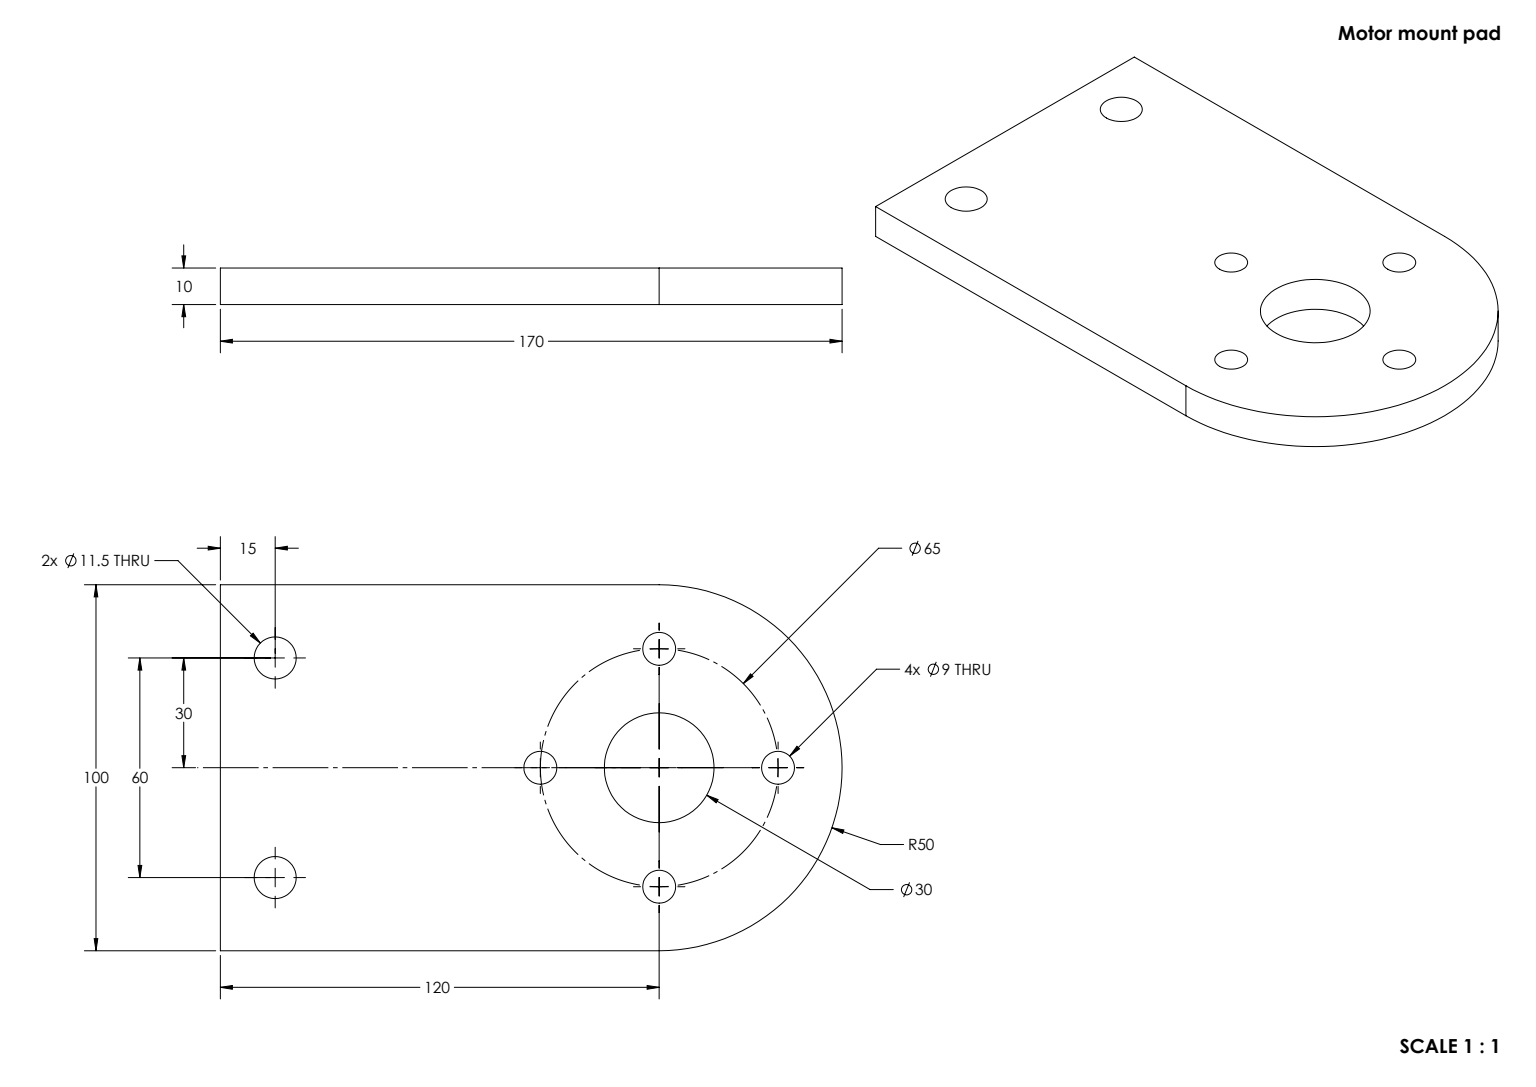
ISO-10303-21;
HEADER;
FILE_DESCRIPTION (('STEP AP214'),
    '1' );
FILE_NAME ('Motor mount pad.step',
    '2026-10-24T15:53:57',
    ( '' ),
    ( '' ),
    'SwSTEP 2.0',
    'SolidWorks 2025',
    '' );
FILE_SCHEMA (( 'AUTOMOTIVE_DESIGN' ));
ENDSEC;

DATA;
#1=CARTESIAN_POINT ( 'NONE',  ( -86.99999999999945999, 120.0000000000003126, 10.00000000000000888 ) ) ;
#4=FACE_BOUND ( 'NONE', #3829, .T. ) ;
#59=DIRECTION ( 'NONE',  ( 3.919652622816902408E-30, 3.944304526105059027E-30, -1.000000000000000000 ) ) ;
#65=LINE ( 'NONE', #1952, #3706 ) ;
#75=DIRECTION ( 'NONE',  ( -3.919652622816902408E-30, -3.944304526105059027E-30, 1.000000000000000000 ) ) ;
#91=DIRECTION ( 'NONE',  ( -3.919652622816902408E-30, -3.944304526105059027E-30, 1.000000000000000000 ) ) ;
#98=EDGE_CURVE ( 'NONE', #113, #2214, #3687, .T. ) ;
#105=UNCERTAINTY_MEASURE_WITH_UNIT (LENGTH_MEASURE( 1.000000000000000082E-05 ), #1753, 'distance_accuracy_value', 'NONE');
#109=DIRECTION ( 'NONE',  ( 3.919652622816902408E-30, 3.944304526105059027E-30, -1.000000000000000000 ) ) ;
#113=VERTEX_POINT ( 'NONE', #6673 ) ;
#117=ORIENTED_EDGE ( 'NONE', *, *, #6294, .F. ) ;
#136=DIRECTION ( 'NONE',  ( -3.919652622816902408E-30, -3.944304526105059027E-30, 1.000000000000000000 ) ) ;
#142=ORIENTED_EDGE ( 'NONE', *, *, #672, .F. ) ;
#165=EDGE_CURVE ( 'NONE', #2264, #3370, #4990, .T. ) ;
#167=CARTESIAN_POINT ( 'NONE',  ( -99.99999999999961631, 120.0000000000001137, 10.00000000000000888 ) ) ;
#175=ORIENTED_EDGE ( 'NONE', *, *, #1489, .T. ) ;
#178=VECTOR ( 'NONE', #4210, 1000.000000000000000 ) ;
#217=VECTOR ( 'NONE', #7393, 1000.000000000000000 ) ;
#237=DIRECTION ( 'NONE',  ( -3.919652622816902408E-30, -3.944304526105059027E-30, 1.000000000000000000 ) ) ;
#246=CARTESIAN_POINT ( 'NONE',  ( -86.99999999999944578, 120.0000000000003126, 10.00000000000000888 ) ) ;
#265=AXIS2_PLACEMENT_3D ( 'NONE', #591, #6694, #3898 ) ;
#270=EDGE_LOOP ( 'NONE', ( #1206, #6558, #6515, #500 ) ) ;
#292=DIRECTION ( 'NONE',  ( 1.000000000000000000, 2.715219353702832714E-15, 0.000000000000000000 ) ) ;
#305=VECTOR ( 'NONE', #380, 1000.000000000000000 ) ;
#306=EDGE_CURVE ( 'NONE', #6636, #757, #6561, .T. ) ;
#320=AXIS2_PLACEMENT_3D ( 'NONE', #2121, #5234, #1317 ) ;
#328=DIRECTION ( 'NONE',  ( 3.919652622816902408E-30, 3.944304526105059027E-30, -1.000000000000000000 ) ) ;
#336=AXIS2_PLACEMENT_3D ( 'NONE', #6289, #351, #5640 ) ;
#337=CARTESIAN_POINT ( 'NONE',  ( 0.000000000000000000, 0.000000000000000000, 10.00000000000000888 ) ) ;
#351=DIRECTION ( 'NONE',  ( -3.919652622816902408E-30, -3.944304526105059027E-30, 1.000000000000000000 ) ) ;
#357=UNCERTAINTY_MEASURE_WITH_UNIT (LENGTH_MEASURE( 1.000000000000000082E-05 ), #6514, 'distance_accuracy_value', 'NONE');
#365=CARTESIAN_POINT ( 'NONE',  ( -99.99999999999972999, 0.000000000000000000, 9.999999999999980460 ) ) ;
#377=ORIENTED_EDGE ( 'NONE', *, *, #1254, .F. ) ;
#380=DIRECTION ( 'NONE',  ( -1.619075244245011540E-15, -1.000000000000000000, 3.747089299799789961E-30 ) ) ;
#381=ORIENTED_EDGE ( 'NONE', *, *, #1415, .T. ) ;
#407=AXIS2_PLACEMENT_3D ( 'NONE', #5310, #7916, #3997 ) ;
#419=EDGE_LOOP ( 'NONE', ( #3396, #2400 ) ) ;
#427=VECTOR ( 'NONE', #3150, 1000.000000000000000 ) ;
#437=DIRECTION ( 'NONE',  ( -1.000000000000000000, -2.775557561562916200E-15, 0.000000000000000000 ) ) ;
#439=ADVANCED_FACE ( 'NONE', ( #590 ), #6765, .F. ) ;
#461=CIRCLE ( 'NONE', #2535, 4.499999999999993783 ) ;
#472=FACE_OUTER_BOUND ( 'NONE', #4653, .T. ) ;
#484=VERTEX_POINT ( 'NONE', #6614 ) ;
#486=ORIENTED_EDGE ( 'NONE', *, *, #7335, .T. ) ;
#492=CARTESIAN_POINT ( 'NONE',  ( -14.24999999999983125, 15.00000000000014211, 10.00000000000000888 ) ) ;
#500=ORIENTED_EDGE ( 'NONE', *, *, #647, .F. ) ;
#506=LINE ( 'NONE', #337, #7415 ) ;
#522=ADVANCED_FACE ( 'NONE', ( #8225 ), #7611, .F. ) ;
#548=CIRCLE ( 'NONE', #5427, 4.499999999999983125 ) ;
#573=DIRECTION ( 'NONE',  ( 3.919652622816902408E-30, 3.944304526105059027E-30, -1.000000000000000000 ) ) ;
#575=CARTESIAN_POINT ( 'NONE',  ( -45.49999999999968026, 87.50000000000036948, -1.942890293094023693E-13 ) ) ;
#590=FACE_OUTER_BOUND ( 'NONE', #2757, .T. ) ;
#591=CARTESIAN_POINT ( 'NONE',  ( -82.49999999999945999, 120.0000000000003268, 10.00000000000000888 ) ) ;
#605=VERTEX_POINT ( 'NONE', #5445 ) ;
#639=PLANE ( 'NONE',  #6979 ) ;
#642=AXIS2_PLACEMENT_3D ( 'NONE', #2902, #2253, #6469 ) ;
#647=EDGE_CURVE ( 'NONE', #2499, #2290, #7527, .T. ) ;
#657=DIRECTION ( 'NONE',  ( 3.919652622816902408E-30, 3.944304526105059027E-30, -1.000000000000000000 ) ) ;
#658=CARTESIAN_POINT ( 'NONE',  ( -82.49999999999945999, 120.0000000000003268, 10.00000000000000888 ) ) ;
#659=AXIS2_PLACEMENT_3D ( 'NONE', #2516, #3903, #4518 ) ;
#672=EDGE_CURVE ( 'NONE', #704, #605, #506, .T. ) ;
#683=VERTEX_POINT ( 'NONE', #6965 ) ;
#694=DIRECTION ( 'NONE',  ( -3.919652622816902408E-30, -3.944304526105059027E-30, 1.000000000000000000 ) ) ;
#704=VERTEX_POINT ( 'NONE', #8349 ) ;
#709=SHAPE_DEFINITION_REPRESENTATION ( #3889, #7270 ) ;
#717=DIRECTION ( 'NONE',  ( 2.775557561562879124E-15, 1.000000000000000000, 3.944304526105070237E-30 ) ) ;
#727=FACE_BOUND ( 'NONE', #4525, .T. ) ;
#739=AXIS2_PLACEMENT_3D ( 'NONE', #6687, #717, #91 ) ;
#751=DIRECTION ( 'NONE',  ( 3.919652622816902408E-30, 3.944304526105059027E-30, -1.000000000000000000 ) ) ;
#757=VERTEX_POINT ( 'NONE', #938 ) ;
#776=DIRECTION ( 'NONE',  ( -3.919652622816902408E-30, -3.944304526105059027E-30, 1.000000000000000000 ) ) ;
#777=DIRECTION ( 'NONE',  ( -1.000000000000000000, 3.498359009886547695E-15, 3.722437396511637546E-30 ) ) ;
#795=EDGE_CURVE ( 'NONE', #2499, #6000, #4916, .T. ) ;
#807=ORIENTED_EDGE ( 'NONE', *, *, #3230, .F. ) ;
#827=CARTESIAN_POINT ( 'NONE',  ( -19.99999999999982947, 15.00000000000012434, 10.00000000000000888 ) ) ;
#886=DIRECTION ( 'NONE',  ( 3.919652622816902408E-30, 3.944304526105059027E-30, -1.000000000000000000 ) ) ;
#910=LINE ( 'NONE', #246, #1515 ) ;
#911=AXIS2_PLACEMENT_3D ( 'NONE', #3791, #7747, #7669 ) ;
#938=CARTESIAN_POINT ( 'NONE',  ( -45.49999999999950262, 152.5000000000003126, -1.942890293094023693E-13 ) ) ;
#952=EDGE_CURVE ( 'NONE', #2264, #484, #8525, .T. ) ;
#989=VECTOR ( 'NONE', #3365, 1000.000000000000000 ) ;
#1000=DIRECTION ( 'NONE',  ( -3.919652622816902408E-30, -3.944304526105059027E-30, 1.000000000000000000 ) ) ;
#1026=AXIS2_PLACEMENT_3D ( 'NONE', #1779, #2283, #6452 ) ;
#1032=EDGE_LOOP ( 'NONE', ( #1487, #8169 ) ) ;
#1104=CARTESIAN_POINT ( 'NONE',  ( -49.99999999999963762, 87.50000000000035527, 9.999999999999786837 ) ) ;
#1107=CARTESIAN_POINT ( 'NONE',  ( -25.74999999999981526, 15.00000000000010836, 10.00000000000000888 ) ) ;
#1119=DIRECTION ( 'NONE',  ( 3.919652622816902408E-30, 3.944304526105059027E-30, -1.000000000000000000 ) ) ;
#1130=CARTESIAN_POINT ( 'NONE',  ( -86.99999999999943157, 120.0000000000003126, -2.775557561562893244E-14 ) ) ;
#1157=CARTESIAN_POINT ( 'NONE',  ( -45.49999999999963052, 87.50000000000036948, 9.999999999999786837 ) ) ;
#1186=ORIENTED_EDGE ( 'NONE', *, *, #2194, .F. ) ;
#1194=CARTESIAN_POINT ( 'NONE',  ( -49.99999999999949551, 152.5000000000003126, -1.942890293094023946E-13 ) ) ;
#1197=DIRECTION ( 'NONE',  ( 1.619075244245011343E-15, 1.000000000000000000, -3.845696912952415736E-30 ) ) ;
#1206=ORIENTED_EDGE ( 'NONE', *, *, #795, .T. ) ;
#1227=EDGE_CURVE ( 'NONE', #4883, #4829, #1432, .T. ) ;
#1254=EDGE_CURVE ( 'NONE', #1438, #6198, #65, .T. ) ;
#1263=ORIENTED_EDGE ( 'NONE', *, *, #2548, .T. ) ;
#1271=ORIENTED_EDGE ( 'NONE', *, *, #7626, .T. ) ;
#1290=FACE_BOUND ( 'NONE', #1032, .T. ) ;
#1299=VECTOR ( 'NONE', #5348, 1000.000000000000000 ) ;
#1302=EDGE_CURVE ( 'NONE', #7833, #7189, #3565, .T. ) ;
#1317=DIRECTION ( 'NONE',  ( 1.000000000000000000, 3.083952846180992055E-15, 0.000000000000000000 ) ) ;
#1323=CYLINDRICAL_SURFACE ( 'NONE', #4448, 4.499999999999990230 ) ;
#1336=FACE_BOUND ( 'NONE', #5358, .T. ) ;
#1346=FACE_OUTER_BOUND ( 'NONE', #4606, .T. ) ;
#1347=ORIENTED_EDGE ( 'NONE', *, *, #4480, .F. ) ;
#1354=CARTESIAN_POINT ( 'NONE',  ( -54.49999999999943867, 152.5000000000003126, 9.999999999999786837 ) ) ;
#1365=ORIENTED_EDGE ( 'NONE', *, *, #7801, .T. ) ;
#1370=CARTESIAN_POINT ( 'NONE',  ( -49.99999999999968026, 87.50000000000035527, -1.942890293094023946E-13 ) ) ;
#1400=AXIS2_PLACEMENT_3D ( 'NONE', #2758, #136, #2163 ) ;
#1404=VECTOR ( 'NONE', #4018, 1000.000000000000000 ) ;
#1415=EDGE_CURVE ( 'NONE', #113, #6113, #8014, .T. ) ;
#1432=LINE ( 'NONE', #6755, #217 ) ;
#1435=CARTESIAN_POINT ( 'NONE',  ( -49.99999999999963762, 87.50000000000035527, 9.999999999999786837 ) ) ;
#1438=VERTEX_POINT ( 'NONE', #6151 ) ;
#1447=ORIENTED_EDGE ( 'NONE', *, *, #7891, .T. ) ;
#1456=DIRECTION ( 'NONE',  ( -1.000000000000000000, -3.083952846180997183E-15, 0.000000000000000000 ) ) ;
#1475=CYLINDRICAL_SURFACE ( 'NONE', #3816, 5.749999999999984013 ) ;
#1484=CARTESIAN_POINT ( 'NONE',  ( -49.99999999999944578, 152.5000000000003126, 9.999999999999786837 ) ) ;
#1487=ORIENTED_EDGE ( 'NONE', *, *, #1489, .F. ) ;
#1489=EDGE_CURVE ( 'NONE', #1438, #4229, #7320, .T. ) ;
#1515=VECTOR ( 'NONE', #2255, 1000.000000000000000 ) ;
#1517=ORIENTED_EDGE ( 'NONE', *, *, #7484, .T. ) ;
#1527=AXIS2_PLACEMENT_3D ( 'NONE', #8120, #6818, #2275 ) ;
#1535=ORIENTED_EDGE ( 'NONE', *, *, #306, .T. ) ;
#1550=CARTESIAN_POINT ( 'NONE',  ( -85.74999999999980105, 15.00000000000010836, 10.00000000000017586 ) ) ;
#1564=ORIENTED_EDGE ( 'NONE', *, *, #8209, .T. ) ;
#1569=LINE ( 'NONE', #2114, #8262 ) ;
#1607=EDGE_LOOP ( 'NONE', ( #1271, #142, #5458, #2317 ) ) ;
#1626=EDGE_CURVE ( 'NONE', #5659, #5363, #2315, .T. ) ;
#1629=CARTESIAN_POINT ( 'NONE',  ( -19.99999999999986855, 15.00000000000012434, 0.000000000000000000 ) ) ;
#1633=DIRECTION ( 'NONE',  ( 3.919652622816902408E-30, 3.944304526105059027E-30, -1.000000000000000000 ) ) ;
#1641=CARTESIAN_POINT ( 'NONE',  ( -54.49999999999948841, 152.5000000000003126, -1.942890293094024198E-13 ) ) ;
#1650=VERTEX_POINT ( 'NONE', #1 ) ;
#1686=VECTOR ( 'NONE', #7251, 1000.000000000000000 ) ;
#1700=CIRCLE ( 'NONE', #5625, 4.499999999999983125 ) ;
#1706=EDGE_LOOP ( 'NONE', ( #2673, #1263, #5085, #5047 ) ) ;
#1711=AXIS2_PLACEMENT_3D ( 'NONE', #8438, #7050, #1197 ) ;
#1732=ORIENTED_EDGE ( 'NONE', *, *, #3516, .T. ) ;
#1752=DIRECTION ( 'NONE',  ( 3.919652622816902408E-30, 3.944304526105059027E-30, -1.000000000000000000 ) ) ;
#1753=( LENGTH_UNIT ( ) NAMED_UNIT ( * ) SI_UNIT ( .MILLI., .METRE. ) );
#1779=CARTESIAN_POINT ( 'NONE',  ( -79.99999999999980105, 15.00000000000012434, 10.00000000000017586 ) ) ;
#1788=CARTESIAN_POINT ( 'NONE',  ( -49.99999999999953815, 120.0000000000003268, 9.999999999999980460 ) ) ;
#1803=DIRECTION ( 'NONE',  ( 3.919652622816902408E-30, 3.944304526105059027E-30, -1.000000000000000000 ) ) ;
#1867=DIRECTION ( 'NONE',  ( -3.919652622816902408E-30, -3.944304526105059027E-30, 1.000000000000000000 ) ) ;
#1881=AXIS2_PLACEMENT_3D ( 'NONE', #2639, #4555, #7817 ) ;
#1883=DIRECTION ( 'NONE',  ( 3.919652622816902408E-30, 3.944304526105059027E-30, -1.000000000000000000 ) ) ;
#1892=AXIS2_PLACEMENT_3D ( 'NONE', #6921, #776, #2136 ) ;
#1903=CIRCLE ( 'NONE', #3449, 5.749999999999985789 ) ;
#1920=DIRECTION ( 'NONE',  ( 3.919652622816902408E-30, 3.944304526105059027E-30, -1.000000000000000000 ) ) ;
#1952=CARTESIAN_POINT ( 'NONE',  ( -21.99999999999954881, 120.0000000000003126, 9.999999999999980460 ) ) ;
#1995=CARTESIAN_POINT ( 'NONE',  ( -49.99999999999968026, 87.50000000000035527, -1.942890293094023946E-13 ) ) ;
#2017=ADVANCED_FACE ( 'NONE', ( #5749 ), #3645, .F. ) ;
#2089=CIRCLE ( 'NONE', #8200, 14.99999999999987388 ) ;
#2102=CARTESIAN_POINT ( 'NONE',  ( -17.49999999999955236, 120.0000000000003268, 9.999999999999980460 ) ) ;
#2110=AXIS2_PLACEMENT_3D ( 'NONE', #3460, #2803, #2846 ) ;
#2114=CARTESIAN_POINT ( 'NONE',  ( -99.99999999999961631, 120.0000000000001137, 10.00000000000000888 ) ) ;
#2116=ORIENTED_EDGE ( 'NONE', *, *, #7710, .F. ) ;
#2121=CARTESIAN_POINT ( 'NONE',  ( -49.99999999999963762, 87.50000000000035527, 9.999999999999786837 ) ) ;
#2136=DIRECTION ( 'NONE',  ( 1.000000000000000000, 3.083952846180994816E-15, -3.821045009664285742E-30 ) ) ;
#2152=ORIENTED_EDGE ( 'NONE', *, *, #7413, .T. ) ;
#2163=DIRECTION ( 'NONE',  ( 1.000000000000000000, 2.715219353702835081E-15, -3.821045009664285041E-30 ) ) ;
#2166=ADVANCED_FACE ( 'NONE', ( #4634 ), #7846, .F. ) ;
#2168=DIRECTION ( 'NONE',  ( 3.919652622816902408E-30, 3.944304526105059027E-30, -1.000000000000000000 ) ) ;
#2169=CIRCLE ( 'NONE', #911, 49.99999999999998579 ) ;
#2173=CARTESIAN_POINT ( 'NONE',  ( -49.99999999999953815, 120.0000000000003268, 9.999999999999980460 ) ) ;
#2175=FACE_OUTER_BOUND ( 'NONE', #5707, .T. ) ;
#2183=LINE ( 'NONE', #4137, #305 ) ;
#2194=EDGE_CURVE ( 'NONE', #6000, #3126, #6856, .T. ) ;
#2214=VERTEX_POINT ( 'NONE', #6727 ) ;
#2216=VERTEX_POINT ( 'NONE', #3412 ) ;
#2244=DIRECTION ( 'NONE',  ( -3.919652622816902408E-30, -3.944304526105059027E-30, 1.000000000000000000 ) ) ;
#2253=DIRECTION ( 'NONE',  ( -3.919652622816902408E-30, -3.944304526105059027E-30, 1.000000000000000000 ) ) ;
#2255=DIRECTION ( 'NONE',  ( 3.919652622816902408E-30, 3.944304526105059027E-30, -1.000000000000000000 ) ) ;
#2262=AXIS2_PLACEMENT_3D ( 'NONE', #5573, #4085, #6270 ) ;
#2264=VERTEX_POINT ( 'NONE', #492 ) ;
#2275=DIRECTION ( 'NONE',  ( 1.000000000000000000, 3.083952846180997183E-15, 0.000000000000000000 ) ) ;
#2283=DIRECTION ( 'NONE',  ( -3.919652622816902408E-30, -3.944304526105059027E-30, 1.000000000000000000 ) ) ;
#2289=CIRCLE ( 'NONE', #2851, 4.499999999999997335 ) ;
#2290=VERTEX_POINT ( 'NONE', #3054 ) ;
#2310=CIRCLE ( 'NONE', #1892, 4.499999999999993783 ) ;
#2315=CIRCLE ( 'NONE', #3842, 4.499999999999990230 ) ;
#2317=ORIENTED_EDGE ( 'NONE', *, *, #2619, .T. ) ;
#2334=CARTESIAN_POINT ( 'NONE',  ( -12.99999999999957723, 120.0000000000003411, 1.763843680267613651E-29 ) ) ;
#2352=CARTESIAN_POINT ( 'NONE',  ( -49.99999999999954525, 120.0000000000003268, 0.000000000000000000 ) ) ;
#2376=DIRECTION ( 'NONE',  ( 3.919652622816902408E-30, 3.944304526105059027E-30, -1.000000000000000000 ) ) ;
#2400=ORIENTED_EDGE ( 'NONE', *, *, #4919, .T. ) ;
#2404=DIRECTION ( 'NONE',  ( -3.919652622816902408E-30, -3.944304526105059027E-30, 1.000000000000000000 ) ) ;
#2430=CARTESIAN_POINT ( 'NONE',  ( 4.059252933785728601E-13, 119.9999999999998863, 10.00000000000000888 ) ) ;
#2499=VERTEX_POINT ( 'NONE', #4932 ) ;
#2512=PLANE ( 'NONE',  #1881 ) ;
#2516=CARTESIAN_POINT ( 'NONE',  ( -79.99999999999972999, 15.00000000000012434, 1.942890293094023946E-13 ) ) ;
#2535=AXIS2_PLACEMENT_3D ( 'NONE', #5424, #6641, #7425 ) ;
#2548=EDGE_CURVE ( 'NONE', #6113, #113, #2089, .T. ) ;
#2553=VECTOR ( 'NONE', #573, 1000.000000000000000 ) ;
#2558=( NAMED_UNIT ( * ) SI_UNIT ( $, .STERADIAN. ) SOLID_ANGLE_UNIT ( ) );
#2577=ORIENTED_EDGE ( 'NONE', *, *, #1227, .F. ) ;
#2619=EDGE_CURVE ( 'NONE', #4829, #2216, #7799, .T. ) ;
#2626=AXIS2_PLACEMENT_3D ( 'NONE', #4703, #6109, #7845 ) ;
#2639=CARTESIAN_POINT ( 'NONE',  ( -49.99999999999954525, 120.0000000000003268, 0.000000000000000000 ) ) ;
#2643=DIRECTION ( 'NONE',  ( 3.821045009664296251E-30, -3.944304526105037307E-30, 1.000000000000000000 ) ) ;
#2650=MECHANICAL_DESIGN_GEOMETRIC_PRESENTATION_REPRESENTATION('',(#3897),#7523);
#2663=EDGE_CURVE ( 'NONE', #2214, #4846, #2922, .T. ) ;
#2673=ORIENTED_EDGE ( 'NONE', *, *, #7484, .F. ) ;
#2705=( GEOMETRIC_REPRESENTATION_CONTEXT ( 3 ) GLOBAL_UNCERTAINTY_ASSIGNED_CONTEXT ( ( #105 ) ) GLOBAL_UNIT_ASSIGNED_CONTEXT ( ( #1753, #6390, #5067 ) ) REPRESENTATION_CONTEXT ( 'NONE', 'WORKASPACE' ) );
#2713=PRODUCT_CONTEXT ( 'NONE', #7696, 'mechanical' ) ;
#2722=CARTESIAN_POINT ( 'NONE',  ( -45.49999999999963762, 87.50000000000036948, 9.999999999999786837 ) ) ;
#2729=ORIENTED_EDGE ( 'NONE', *, *, #2619, .F. ) ;
#2757=EDGE_LOOP ( 'NONE', ( #175, #5288, #7117, #377 ) ) ;
#2758=CARTESIAN_POINT ( 'NONE',  ( -19.99999999999986855, 15.00000000000012434, 0.000000000000000000 ) ) ;
#2780=VECTOR ( 'NONE', #3799, 1000.000000000000000 ) ;
#2796=ORIENTED_EDGE ( 'NONE', *, *, #2548, .F. ) ;
#2803=DIRECTION ( 'NONE',  ( -3.919652622816902408E-30, -3.944304526105059027E-30, 1.000000000000000000 ) ) ;
#2806=ORIENTED_EDGE ( 'NONE', *, *, #4919, .F. ) ;
#2846=DIRECTION ( 'NONE',  ( 1.000000000000000000, 3.083952846180994816E-15, -3.821045009664285742E-30 ) ) ;
#2848=EDGE_LOOP ( 'NONE', ( #2881, #1447, #3011, #7362 ) ) ;
#2851=AXIS2_PLACEMENT_3D ( 'NONE', #1435, #694, #8099 ) ;
#2864=CARTESIAN_POINT ( 'NONE',  ( -14.24999999999984368, 15.00000000000014211, 10.00000000000000888 ) ) ;
#2865=CARTESIAN_POINT ( 'NONE',  ( -49.99999999999944578, 152.5000000000003126, 9.999999999999786837 ) ) ;
#2867=DIRECTION ( 'NONE',  ( 3.919652622816902408E-30, 3.944304526105059027E-30, -1.000000000000000000 ) ) ;
#2881=ORIENTED_EDGE ( 'NONE', *, *, #7184, .F. ) ;
#2900=CYLINDRICAL_SURFACE ( 'NONE', #2262, 5.749999999999991118 ) ;
#2902=CARTESIAN_POINT ( 'NONE',  ( -17.49999999999955236, 120.0000000000003268, 9.999999999999980460 ) ) ;
#2921=CIRCLE ( 'NONE', #1400, 5.749999999999985789 ) ;
#2922=CIRCLE ( 'NONE', #6406, 14.99999999999987388 ) ;
#2940=ORIENTED_EDGE ( 'NONE', *, *, #4022, .F. ) ;
#2942=ADVANCED_FACE ( 'NONE', ( #4608 ), #5117, .F. ) ;
#2953=VERTEX_POINT ( 'NONE', #6403 ) ;
#2963=MANIFOLD_SOLID_BREP ( 'Boss-Extrude1', #7516 ) ;
#2998=ORIENTED_EDGE ( 'NONE', *, *, #8586, .F. ) ;
#3011=ORIENTED_EDGE ( 'NONE', *, *, #7073, .T. ) ;
#3024=SHAPE_REPRESENTATION_RELATIONSHIP ( 'NONE' , 'NONE' ,  #7270, #3221 ) ;
#3043=ADVANCED_FACE ( 'NONE', ( #8134, #727, #4738, #2175, #4822, #1336, #1290, #3948 ), #639, .T. ) ;
#3044=CIRCLE ( 'NONE', #4155, 4.499999999999983125 ) ;
#3054=CARTESIAN_POINT ( 'NONE',  ( -85.74999999999972999, 15.00000000000010836, 1.942890293094023693E-13 ) ) ;
#3066=LINE ( 'NONE', #7118, #3329 ) ;
#3091=AXIS2_PLACEMENT_3D ( 'NONE', #2102, #657, #8020 ) ;
#3093=LINE ( 'NONE', #3873, #4209 ) ;
#3110=CIRCLE ( 'NONE', #4628, 14.99999999999987388 ) ;
#3123=FACE_OUTER_BOUND ( 'NONE', #6717, .T. ) ;
#3126=VERTEX_POINT ( 'NONE', #4050 ) ;
#3135=DIRECTION ( 'NONE',  ( 3.919652622816902408E-30, 3.944304526105059027E-30, -1.000000000000000000 ) ) ;
#3150=DIRECTION ( 'NONE',  ( 1.000000000000000000, 2.775557561562898056E-15, -3.821045009664285041E-30 ) ) ;
#3162=DIRECTION ( 'NONE',  ( 1.000000000000000000, 0.000000000000000000, -5.478200730701491345E-30 ) ) ;
#3164=FACE_BOUND ( 'NONE', #7637, .T. ) ;
#3169=EDGE_LOOP ( 'NONE', ( #381, #1517, #7092, #4001 ) ) ;
#3183=AXIS2_PLACEMENT_3D ( 'NONE', #4392, #2376, #7732 ) ;
#3195=PRODUCT ( 'Motor mount pad', 'Motor mount pad', '', ( #2713 ) ) ;
#3200=LINE ( 'NONE', #4552, #1686 ) ;
#3216=DIRECTION ( 'NONE',  ( 1.000000000000000000, 0.000000000000000000, 0.000000000000000000 ) ) ;
#3221=ADVANCED_BREP_SHAPE_REPRESENTATION ( '', ( #2963, #7563 ), #2705 ) ;
#3230=EDGE_CURVE ( 'NONE', #6497, #2216, #2183, .T. ) ;
#3232=FACE_OUTER_BOUND ( 'NONE', #4254, .T. ) ;
#3260=ORIENTED_EDGE ( 'NONE', *, *, #7184, .T. ) ;
#3288=CARTESIAN_POINT ( 'NONE',  ( -49.99999999999953815, 120.0000000000003268, 9.999999999999980460 ) ) ;
#3301=DIRECTION ( 'NONE',  ( 1.000000000000000000, 2.775557561562914622E-15, 0.000000000000000000 ) ) ;
#3329=VECTOR ( 'NONE', #4417, 1000.000000000000000 ) ;
#3330=FACE_OUTER_BOUND ( 'NONE', #3585, .T. ) ;
#3347=DIRECTION ( 'NONE',  ( 3.919652622816902408E-30, 3.944304526105059027E-30, -1.000000000000000000 ) ) ;
#3365=DIRECTION ( 'NONE',  ( 3.498359009886546906E-15, 1.000000000000000000, -3.747089299799789961E-30 ) ) ;
#3370=VERTEX_POINT ( 'NONE', #5245 ) ;
#3371=DIRECTION ( 'NONE',  ( -3.919652622816902408E-30, -3.944304526105059027E-30, 1.000000000000000000 ) ) ;
#3393=CYLINDRICAL_SURFACE ( 'NONE', #2626, 5.749999999999984013 ) ;
#3396=ORIENTED_EDGE ( 'NONE', *, *, #7943, .T. ) ;
#3412=CARTESIAN_POINT ( 'NONE',  ( -99.99999999999972999, 0.000000000000000000, -2.775557561562891351E-14 ) ) ;
#3416=PLANE ( 'NONE',  #739 ) ;
#3430=EDGE_CURVE ( 'NONE', #484, #4252, #7078, .T. ) ;
#3435=AXIS2_PLACEMENT_3D ( 'NONE', #7386, #2244, #4122 ) ;
#3441=ORIENTED_EDGE ( 'NONE', *, *, #5342, .F. ) ;
#3449=AXIS2_PLACEMENT_3D ( 'NONE', #1629, #75, #3486 ) ;
#3460=CARTESIAN_POINT ( 'NONE',  ( -17.49999999999958078, 120.0000000000003268, 0.000000000000000000 ) ) ;
#3479=ORIENTED_EDGE ( 'NONE', *, *, #8209, .F. ) ;
#3486=DIRECTION ( 'NONE',  ( 1.000000000000000000, 2.715219353702835081E-15, -3.821045009664285041E-30 ) ) ;
#3512=DIRECTION ( 'NONE',  ( 1.000000000000000000, 0.000000000000000000, 0.000000000000000000 ) ) ;
#3516=EDGE_CURVE ( 'NONE', #4229, #1438, #461, .T. ) ;
#3517=CARTESIAN_POINT ( 'NONE',  ( 0.000000000000000000, 0.000000000000000000, 10.00000000000000888 ) ) ;
#3537=ORIENTED_EDGE ( 'NONE', *, *, #6441, .T. ) ;
#3542=PRODUCT_DEFINITION_FORMATION_WITH_SPECIFIED_SOURCE ( 'ANY', '', #3195, .NOT_KNOWN. ) ;
#3561=ADVANCED_FACE ( 'NONE', ( #6734 ), #3416, .F. ) ;
#3565=CIRCLE ( 'NONE', #4679, 4.499999999999997335 ) ;
#3566=DIRECTION ( 'NONE',  ( -3.498359009886547695E-15, -1.000000000000000000, 3.845696912952415736E-30 ) ) ;
#3573=EDGE_CURVE ( 'NONE', #4804, #7222, #7823, .T. ) ;
#3585=EDGE_LOOP ( 'NONE', ( #1186, #8320, #7688, #5000 ) ) ;
#3605=DIRECTION ( 'NONE',  ( 1.000000000000000000, 2.775557561562914622E-15, -3.821045009664285041E-30 ) ) ;
#3610=CYLINDRICAL_SURFACE ( 'NONE', #6508, 4.499999999999983125 ) ;
#3617=VECTOR ( 'NONE', #1119, 1000.000000000000000 ) ;
#3645=CYLINDRICAL_SURFACE ( 'NONE', #8073, 4.499999999999997335 ) ;
#3654=DIRECTION ( 'NONE',  ( 1.000000000000000000, 2.775557561562914622E-15, 0.000000000000000000 ) ) ;
#3687=LINE ( 'NONE', #5271, #8092 ) ;
#3706=VECTOR ( 'NONE', #109, 1000.000000000000000 ) ;
#3727=DIRECTION ( 'NONE',  ( -1.000000000000000000, -3.083952846180992055E-15, 0.000000000000000000 ) ) ;
#3730=ORIENTED_EDGE ( 'NONE', *, *, #795, .F. ) ;
#3765=EDGE_CURVE ( 'NONE', #4846, #2214, #3110, .T. ) ;
#3782=ORIENTED_EDGE ( 'NONE', *, *, #1415, .F. ) ;
#3785=ADVANCED_FACE ( 'NONE', ( #4207 ), #2900, .F. ) ;
#3791=CARTESIAN_POINT ( 'NONE',  ( -49.99999999999954525, 120.0000000000003268, 0.000000000000000000 ) ) ;
#3799=DIRECTION ( 'NONE',  ( 3.919652622816902408E-30, 3.944304526105059027E-30, -1.000000000000000000 ) ) ;
#3816=AXIS2_PLACEMENT_3D ( 'NONE', #827, #3347, #4490 ) ;
#3817=CARTESIAN_POINT ( 'NONE',  ( -54.49999999999968736, 87.50000000000034106, -1.942890293094024198E-13 ) ) ;
#3820=ORIENTED_EDGE ( 'NONE', *, *, #8339, .F. ) ;
#3825=CARTESIAN_POINT ( 'NONE',  ( -19.99999999999982947, 15.00000000000012434, 10.00000000000000888 ) ) ;
#3829=EDGE_LOOP ( 'NONE', ( #6157, #5735 ) ) ;
#3830=FACE_OUTER_BOUND ( 'NONE', #2848, .T. ) ;
#3839=LINE ( 'NONE', #2430, #2553 ) ;
#3842=AXIS2_PLACEMENT_3D ( 'NONE', #5804, #5110, #4389 ) ;
#3856=CARTESIAN_POINT ( 'NONE',  ( -49.99999999999953815, 120.0000000000003268, 9.999999999999980460 ) ) ;
#3873=CARTESIAN_POINT ( 'NONE',  ( -12.99999999999956124, 120.0000000000003411, 9.999999999999980460 ) ) ;
#3874=DIRECTION ( 'NONE',  ( 3.919652622816902408E-30, 3.944304526105059027E-30, -1.000000000000000000 ) ) ;
#3884=LINE ( 'NONE', #5379, #989 ) ;
#3889=PRODUCT_DEFINITION_SHAPE ( 'NONE', 'NONE',  #4926 ) ;
#3897=STYLED_ITEM('',(#8656),#2963);
#3898=DIRECTION ( 'NONE',  ( 1.000000000000000000, 3.083952846180997183E-15, 0.000000000000000000 ) ) ;
#3903=DIRECTION ( 'NONE',  ( -3.919652622816902408E-30, -3.944304526105059027E-30, 1.000000000000000000 ) ) ;
#3943=FACE_BOUND ( 'NONE', #419, .T. ) ;
#3948=FACE_BOUND ( 'NONE', #7617, .T. ) ;
#3968=CARTESIAN_POINT ( 'NONE',  ( -54.49999999999963762, 87.50000000000034106, 9.999999999999786837 ) ) ;
#3979=DIRECTION ( 'NONE',  ( 3.919652622816902408E-30, 3.944304526105059027E-30, -1.000000000000000000 ) ) ;
#3980=ORIENTED_EDGE ( 'NONE', *, *, #3573, .T. ) ;
#3990=DIRECTION ( 'NONE',  ( 1.000000000000000000, 2.775557561562898056E-15, -3.821045009664285041E-30 ) ) ;
#3997=DIRECTION ( 'NONE',  ( 1.000000000000000000, 2.775557561562892140E-15, 0.000000000000000000 ) ) ;
#4001=ORIENTED_EDGE ( 'NONE', *, *, #98, .F. ) ;
#4008=DIRECTION ( 'NONE',  ( 1.000000000000000000, 0.000000000000000000, 0.000000000000000000 ) ) ;
#4018=DIRECTION ( 'NONE',  ( 3.919652622816902408E-30, 3.944304526105059027E-30, -1.000000000000000000 ) ) ;
#4022=EDGE_CURVE ( 'NONE', #7189, #7833, #5053, .T. ) ;
#4025=ORIENTED_EDGE ( 'NONE', *, *, #4549, .F. ) ;
#4050=CARTESIAN_POINT ( 'NONE',  ( -74.24999999999971578, 15.00000000000014211, 1.942890293094024198E-13 ) ) ;
#4085=DIRECTION ( 'NONE',  ( 3.919652622816902408E-30, 3.944304526105059027E-30, -1.000000000000000000 ) ) ;
#4100=DIRECTION ( 'NONE',  ( -3.919652622816902408E-30, -3.944304526105059027E-30, 1.000000000000000000 ) ) ;
#4113=AXIS2_PLACEMENT_3D ( 'NONE', #8138, #1000, #3654 ) ;
#4122=DIRECTION ( 'NONE',  ( 1.000000000000000000, 2.715219353702832714E-15, -4.287287528375070588E-30 ) ) ;
#4137=CARTESIAN_POINT ( 'NONE',  ( -99.99999999999972999, 0.000000000000000000, -2.775557561562891351E-14 ) ) ;
#4143=ADVANCED_FACE ( 'NONE', ( #8127 ), #5472, .F. ) ;
#4146=ORIENTED_EDGE ( 'NONE', *, *, #6773, .F. ) ;
#4155=AXIS2_PLACEMENT_3D ( 'NONE', #7829, #1867, #3216 ) ;
#4160=CYLINDRICAL_SURFACE ( 'NONE', #8560, 49.99999999999999289 ) ;
#4161=ORIENTED_EDGE ( 'NONE', *, *, #952, .F. ) ;
#4200=DIRECTION ( 'NONE',  ( 1.000000000000000000, 0.000000000000000000, -5.478200730701491345E-30 ) ) ;
#4203=CARTESIAN_POINT ( 'NONE',  ( 0.000000000000000000, 0.000000000000000000, 0.000000000000000000 ) ) ;
#4207=FACE_OUTER_BOUND ( 'NONE', #270, .T. ) ;
#4209=VECTOR ( 'NONE', #1920, 1000.000000000000000 ) ;
#4210=DIRECTION ( 'NONE',  ( 3.919652622816902408E-30, 3.944304526105059027E-30, -1.000000000000000000 ) ) ;
#4229=VERTEX_POINT ( 'NONE', #7681 ) ;
#4252=VERTEX_POINT ( 'NONE', #4413 ) ;
#4254=EDGE_LOOP ( 'NONE', ( #486, #3260, #4146, #6165 ) ) ;
#4314=ORIENTED_EDGE ( 'NONE', *, *, #3573, .F. ) ;
#4332=EDGE_LOOP ( 'NONE', ( #7723, #6024, #4944, #2806 ) ) ;
#4346=LINE ( 'NONE', #7012, #3617 ) ;
#4389=DIRECTION ( 'NONE',  ( 1.000000000000000000, 3.083952846180997183E-15, -4.108650548026112028E-30 ) ) ;
#4392=CARTESIAN_POINT ( 'NONE',  ( -49.99999999999944578, 152.5000000000003126, 9.999999999999786837 ) ) ;
#4413=CARTESIAN_POINT ( 'NONE',  ( -25.74999999999986855, 15.00000000000010836, -2.234078735489214329E-29 ) ) ;
#4417=DIRECTION ( 'NONE',  ( 3.919652622816902408E-30, 3.944304526105059027E-30, -1.000000000000000000 ) ) ;
#4429=VERTEX_POINT ( 'NONE', #5206 ) ;
#4439=CIRCLE ( 'NONE', #265, 4.499999999999990230 ) ;
#4448=AXIS2_PLACEMENT_3D ( 'NONE', #5921, #3979, #1456 ) ;
#4457=CYLINDRICAL_SURFACE ( 'NONE', #4864, 4.499999999999997335 ) ;
#4480=EDGE_CURVE ( 'NONE', #683, #4429, #3839, .T. ) ;
#4487=ORIENTED_EDGE ( 'NONE', *, *, #7801, .F. ) ;
#4490=DIRECTION ( 'NONE',  ( -1.000000000000000000, -2.715219353702835870E-15, 0.000000000000000000 ) ) ;
#4518=DIRECTION ( 'NONE',  ( 1.000000000000000000, 2.715219353702832714E-15, -4.287287528375070588E-30 ) ) ;
#4525=EDGE_LOOP ( 'NONE', ( #3782, #2796 ) ) ;
#4542=ORIENTED_EDGE ( 'NONE', *, *, #1302, .F. ) ;
#4549=EDGE_CURVE ( 'NONE', #4883, #6497, #1569, .T. ) ;
#4552=CARTESIAN_POINT ( 'NONE',  ( 0.000000000000000000, 0.000000000000000000, 10.00000000000000888 ) ) ;
#4555=DIRECTION ( 'NONE',  ( 3.821045009664296251E-30, -3.944304526105037307E-30, 1.000000000000000000 ) ) ;
#4570=ORIENTED_EDGE ( 'NONE', *, *, #8586, .T. ) ;
#4598=DIRECTION ( 'NONE',  ( 1.000000000000000000, 3.083952846180992055E-15, -5.478200730701473829E-30 ) ) ;
#4606=EDGE_LOOP ( 'NONE', ( #6823, #8173, #5545, #7431 ) ) ;
#4608=FACE_OUTER_BOUND ( 'NONE', #3169, .T. ) ;
#4628=AXIS2_PLACEMENT_3D ( 'NONE', #4905, #5624, #3605 ) ;
#4634=FACE_OUTER_BOUND ( 'NONE', #8001, .T. ) ;
#4645=EDGE_LOOP ( 'NONE', ( #3537, #5892, #6391, #3820 ) ) ;
#4652=CARTESIAN_POINT ( 'NONE',  ( -54.49999999999963052, 87.50000000000034106, 9.999999999999786837 ) ) ;
#4653=EDGE_LOOP ( 'NONE', ( #2116, #4978, #7483, #6367 ) ) ;
#4659=DIRECTION ( 'NONE',  ( 1.000000000000000000, 3.083952846180992055E-15, -5.478200730701473829E-30 ) ) ;
#4679=AXIS2_PLACEMENT_3D ( 'NONE', #1995, #7261, #4659 ) ;
#4703=CARTESIAN_POINT ( 'NONE',  ( -19.99999999999982947, 15.00000000000012434, 10.00000000000000888 ) ) ;
#4738=FACE_BOUND ( 'NONE', #6008, .T. ) ;
#4775=VERTEX_POINT ( 'NONE', #1354 ) ;
#4789=FACE_OUTER_BOUND ( 'NONE', #4332, .T. ) ;
#4804=VERTEX_POINT ( 'NONE', #3968 ) ;
#4810=ADVANCED_FACE ( 'NONE', ( #3830 ), #7794, .F. ) ;
#4822=FACE_BOUND ( 'NONE', #6103, .T. ) ;
#4829=VERTEX_POINT ( 'NONE', #5065 ) ;
#4846=VERTEX_POINT ( 'NONE', #7925 ) ;
#4864=AXIS2_PLACEMENT_3D ( 'NONE', #1104, #1752, #3727 ) ;
#4883=VERTEX_POINT ( 'NONE', #167 ) ;
#4905=CARTESIAN_POINT ( 'NONE',  ( -49.99999999999954525, 120.0000000000003268, 0.000000000000000000 ) ) ;
#4916=CIRCLE ( 'NONE', #1026, 5.749999999999991118 ) ;
#4919=EDGE_CURVE ( 'NONE', #3370, #4252, #1903, .T. ) ;
#4926=PRODUCT_DEFINITION ( 'UNKNOWN', '', #3542, #8548 ) ;
#4932=CARTESIAN_POINT ( 'NONE',  ( -85.74999999999981526, 15.00000000000010836, 10.00000000000017586 ) ) ;
#4942=LINE ( 'NONE', #5478, #8214 ) ;
#4944=ORIENTED_EDGE ( 'NONE', *, *, #3430, .T. ) ;
#4955=ORIENTED_EDGE ( 'NONE', *, *, #7992, .F. ) ;
#4975=VERTEX_POINT ( 'NONE', #6159 ) ;
#4978=ORIENTED_EDGE ( 'NONE', *, *, #6832, .T. ) ;
#4990=LINE ( 'NONE', #2864, #6431 ) ;
#5000=ORIENTED_EDGE ( 'NONE', *, *, #5598, .F. ) ;
#5013=DIRECTION ( 'NONE',  ( 1.000000000000000000, 2.775557561562914622E-15, -3.821045009664285041E-30 ) ) ;
#5016=EDGE_CURVE ( 'NONE', #2290, #3126, #5537, .T. ) ;
#5022=FACE_OUTER_BOUND ( 'NONE', #5785, .T. ) ;
#5023=ORIENTED_EDGE ( 'NONE', *, *, #7992, .T. ) ;
#5026=ORIENTED_EDGE ( 'NONE', *, *, #4549, .T. ) ;
#5044=DIRECTION ( 'NONE',  ( 1.000000000000000000, 2.715219353702835081E-15, 0.000000000000000000 ) ) ;
#5047=ORIENTED_EDGE ( 'NONE', *, *, #3765, .F. ) ;
#5053=CIRCLE ( 'NONE', #5782, 4.499999999999997335 ) ;
#5054=CARTESIAN_POINT ( 'NONE',  ( -34.99999999999963052, 120.0000000000003695, 9.999999999999980460 ) ) ;
#5065=CARTESIAN_POINT ( 'NONE',  ( -99.99999999999972999, 0.000000000000000000, 9.999999999999980460 ) ) ;
#5067=( NAMED_UNIT ( * ) SI_UNIT ( $, .STERADIAN. ) SOLID_ANGLE_UNIT ( ) );
#5085=ORIENTED_EDGE ( 'NONE', *, *, #98, .T. ) ;
#5110=DIRECTION ( 'NONE',  ( -3.919652622816902408E-30, -3.944304526105059027E-30, 1.000000000000000000 ) ) ;
#5117=CYLINDRICAL_SURFACE ( 'NONE', #6686, 14.99999999999986677 ) ;
#5146=DIRECTION ( 'NONE',  ( 3.919652622816902408E-30, 3.944304526105059027E-30, -1.000000000000000000 ) ) ;
#5171=ORIENTED_EDGE ( 'NONE', *, *, #4480, .T. ) ;
#5206=CARTESIAN_POINT ( 'NONE',  ( 4.059252933785728601E-13, 119.9999999999998863, 0.000000000000000000 ) ) ;
#5234=DIRECTION ( 'NONE',  ( -3.919652622816902408E-30, -3.944304526105059027E-30, 1.000000000000000000 ) ) ;
#5245=CARTESIAN_POINT ( 'NONE',  ( -14.24999999999986855, 15.00000000000014211, 2.234078735489191628E-29 ) ) ;
#5246=EDGE_LOOP ( 'NONE', ( #1365, #1347, #7194, #6728 ) ) ;
#5256=ORIENTED_EDGE ( 'NONE', *, *, #6832, .F. ) ;
#5271=CARTESIAN_POINT ( 'NONE',  ( -64.99999999999940314, 120.0000000000002842, 9.999999999999980460 ) ) ;
#5288=ORIENTED_EDGE ( 'NONE', *, *, #6294, .T. ) ;
#5298=CARTESIAN_POINT ( 'NONE',  ( -79.99999999999980105, 15.00000000000012434, 10.00000000000017586 ) ) ;
#5310=CARTESIAN_POINT ( 'NONE',  ( -49.99999999999953815, 120.0000000000003268, 9.999999999999980460 ) ) ;
#5342=EDGE_CURVE ( 'NONE', #4429, #6497, #2169, .T. ) ;
#5348=DIRECTION ( 'NONE',  ( 3.919652622816902408E-30, 3.944304526105059027E-30, -1.000000000000000000 ) ) ;
#5358=EDGE_LOOP ( 'NONE', ( #6620, #5256 ) ) ;
#5363=VERTEX_POINT ( 'NONE', #1130 ) ;
#5377=DIRECTION ( 'NONE',  ( -1.000000000000000000, -3.083952846180994816E-15, 0.000000000000000000 ) ) ;
#5379=CARTESIAN_POINT ( 'NONE',  ( 0.000000000000000000, 0.000000000000000000, 0.000000000000000000 ) ) ;
#5382=CIRCLE ( 'NONE', #3435, 5.749999999999991118 ) ;
#5388=CARTESIAN_POINT ( 'NONE',  ( -74.24999999999980105, 15.00000000000014211, 10.00000000000017586 ) ) ;
#5400=CIRCLE ( 'NONE', #6056, 5.749999999999991118 ) ;
#5424=CARTESIAN_POINT ( 'NONE',  ( -17.49999999999955236, 120.0000000000003268, 9.999999999999980460 ) ) ;
#5427=AXIS2_PLACEMENT_3D ( 'NONE', #6827, #237, #4200 ) ;
#5445=CARTESIAN_POINT ( 'NONE',  ( 0.000000000000000000, 0.000000000000000000, 0.000000000000000000 ) ) ;
#5458=ORIENTED_EDGE ( 'NONE', *, *, #7040, .F. ) ;
#5463=CARTESIAN_POINT ( 'NONE',  ( -74.24999999999981526, 15.00000000000014211, 10.00000000000017586 ) ) ;
#5472=CYLINDRICAL_SURFACE ( 'NONE', #5907, 14.99999999999986677 ) ;
#5478=CARTESIAN_POINT ( 'NONE',  ( -34.99999999999966604, 120.0000000000003695, 9.999999999999980460 ) ) ;
#5501=EDGE_LOOP ( 'NONE', ( #1535, #2152 ) ) ;
#5532=ADVANCED_FACE ( 'NONE', ( #6014, #8598, #3943, #6605, #4, #3164, #5845, #8472 ), #2512, .F. ) ;
#5537=CIRCLE ( 'NONE', #659, 5.749999999999991118 ) ;
#5545=ORIENTED_EDGE ( 'NONE', *, *, #7943, .F. ) ;
#5573=CARTESIAN_POINT ( 'NONE',  ( -79.99999999999980105, 15.00000000000012434, 10.00000000000017586 ) ) ;
#5580=CIRCLE ( 'NONE', #1527, 4.499999999999990230 ) ;
#5595=ORIENTED_EDGE ( 'NONE', *, *, #7335, .F. ) ;
#5598=EDGE_CURVE ( 'NONE', #3126, #2290, #5382, .T. ) ;
#5616=ADVANCED_FACE ( 'NONE', ( #8172 ), #4160, .T. ) ;
#5624=DIRECTION ( 'NONE',  ( -3.919652622816902408E-30, -3.944304526105059027E-30, 1.000000000000000000 ) ) ;
#5625=AXIS2_PLACEMENT_3D ( 'NONE', #1484, #4100, #4008 ) ;
#5640=DIRECTION ( 'NONE',  ( 1.000000000000000000, 2.715219353702835081E-15, 0.000000000000000000 ) ) ;
#5653=EDGE_LOOP ( 'NONE', ( #8398, #4025, #7945, #5171 ) ) ;
#5659=VERTEX_POINT ( 'NONE', #8005 ) ;
#5705=EDGE_CURVE ( 'NONE', #6198, #7037, #2310, .T. ) ;
#5707=EDGE_LOOP ( 'NONE', ( #7227, #7864, #7551, #7540 ) ) ;
#5708=LINE ( 'NONE', #7760, #427 ) ;
#5714=EDGE_LOOP ( 'NONE', ( #4314, #3479 ) ) ;
#5734=CARTESIAN_POINT ( 'NONE',  ( -82.49999999999941735, 120.0000000000003268, -2.775557561562891351E-14 ) ) ;
#5735=ORIENTED_EDGE ( 'NONE', *, *, #3765, .T. ) ;
#5749=FACE_OUTER_BOUND ( 'NONE', #8578, .T. ) ;
#5782=AXIS2_PLACEMENT_3D ( 'NONE', #1370, #3371, #4598 ) ;
#5785=EDGE_LOOP ( 'NONE', ( #3980, #7158, #2940, #2998 ) ) ;
#5804=CARTESIAN_POINT ( 'NONE',  ( -82.49999999999941735, 120.0000000000003268, -2.775557561562891351E-14 ) ) ;
#5808=PLANE ( 'NONE',  #1711 ) ;
#5830=DIRECTION ( 'NONE',  ( -1.000000000000000000, -3.083952846180992055E-15, 0.000000000000000000 ) ) ;
#5845=FACE_BOUND ( 'NONE', #6264, .T. ) ;
#5851=CIRCLE ( 'NONE', #6944, 5.749999999999985789 ) ;
#5855=CIRCLE ( 'NONE', #8191, 4.499999999999990230 ) ;
#5879=LINE ( 'NONE', #2722, #1404 ) ;
#5881=ORIENTED_EDGE ( 'NONE', *, *, #5016, .T. ) ;
#5892=ORIENTED_EDGE ( 'NONE', *, *, #7710, .T. ) ;
#5893=DIRECTION ( 'NONE',  ( 3.919652622816902408E-30, 3.944304526105059027E-30, -1.000000000000000000 ) ) ;
#5907=AXIS2_PLACEMENT_3D ( 'NONE', #6784, #2168, #7473 ) ;
#5914=ORIENTED_EDGE ( 'NONE', *, *, #1302, .T. ) ;
#5921=CARTESIAN_POINT ( 'NONE',  ( -82.49999999999945999, 120.0000000000003268, 10.00000000000000888 ) ) ;
#5938=ADVANCED_FACE ( 'NONE', ( #3330 ), #7949, .F. ) ;
#6000=VERTEX_POINT ( 'NONE', #5388 ) ;
#6008=EDGE_LOOP ( 'NONE', ( #6258, #4161 ) ) ;
#6012=DIRECTION ( 'NONE',  ( 3.919652622816902408E-30, 3.944304526105059027E-30, -1.000000000000000000 ) ) ;
#6014=FACE_OUTER_BOUND ( 'NONE', #6286, .T. ) ;
#6024=ORIENTED_EDGE ( 'NONE', *, *, #952, .T. ) ;
#6038=ORIENTED_EDGE ( 'NONE', *, *, #7761, .F. ) ;
#6043=EDGE_CURVE ( 'NONE', #704, #683, #3200, .T. ) ;
#6056=AXIS2_PLACEMENT_3D ( 'NONE', #8229, #7573, #292 ) ;
#6072=ORIENTED_EDGE ( 'NONE', *, *, #4022, .T. ) ;
#6103=EDGE_LOOP ( 'NONE', ( #3730, #7066 ) ) ;
#6109=DIRECTION ( 'NONE',  ( 3.919652622816902408E-30, 3.944304526105059027E-30, -1.000000000000000000 ) ) ;
#6113=VERTEX_POINT ( 'NONE', #5054 ) ;
#6133=ORIENTED_EDGE ( 'NONE', *, *, #5705, .T. ) ;
#6151=CARTESIAN_POINT ( 'NONE',  ( -21.99999999999955946, 120.0000000000003126, 9.999999999999980460 ) ) ;
#6153=CARTESIAN_POINT ( 'NONE',  ( 0.000000000000000000, 0.000000000000000000, 10.00000000000000888 ) ) ;
#6157=ORIENTED_EDGE ( 'NONE', *, *, #2663, .T. ) ;
#6159=CARTESIAN_POINT ( 'NONE',  ( -45.49999999999945999, 152.5000000000003126, 9.999999999999786837 ) ) ;
#6165=ORIENTED_EDGE ( 'NONE', *, *, #7073, .F. ) ;
#6197=CARTESIAN_POINT ( 'NONE',  ( -54.49999999999943157, 152.5000000000003126, 9.999999999999786837 ) ) ;
#6198=VERTEX_POINT ( 'NONE', #6379 ) ;
#6238=AXIS2_PLACEMENT_3D ( 'NONE', #3517, #777, #3566 ) ;
#6258=ORIENTED_EDGE ( 'NONE', *, *, #6725, .F. ) ;
#6264=EDGE_LOOP ( 'NONE', ( #6072, #5914 ) ) ;
#6270=DIRECTION ( 'NONE',  ( -1.000000000000000000, -2.715219353702832714E-15, 0.000000000000000000 ) ) ;
#6280=VECTOR ( 'NONE', #886, 1000.000000000000000 ) ;
#6286=EDGE_LOOP ( 'NONE', ( #7289, #807, #3441, #4487 ) ) ;
#6289=CARTESIAN_POINT ( 'NONE',  ( -19.99999999999982947, 15.00000000000012434, 10.00000000000000888 ) ) ;
#6294=EDGE_CURVE ( 'NONE', #4229, #7037, #3093, .T. ) ;
#6322=DIRECTION ( 'NONE',  ( -1.000000000000000000, 0.000000000000000000, 0.000000000000000000 ) ) ;
#6346=ORIENTED_EDGE ( 'NONE', *, *, #1254, .T. ) ;
#6367=ORIENTED_EDGE ( 'NONE', *, *, #7413, .F. ) ;
#6379=CARTESIAN_POINT ( 'NONE',  ( -21.99999999999958433, 120.0000000000003126, -1.763843680267613651E-29 ) ) ;
#6390=( NAMED_UNIT ( * ) PLANE_ANGLE_UNIT ( ) SI_UNIT ( $, .RADIAN. ) );
#6391=ORIENTED_EDGE ( 'NONE', *, *, #306, .F. ) ;
#6403=CARTESIAN_POINT ( 'NONE',  ( -77.99999999999945999, 120.0000000000003411, 10.00000000000000888 ) ) ;
#6406=AXIS2_PLACEMENT_3D ( 'NONE', #2352, #7157, #5013 ) ;
#6431=VECTOR ( 'NONE', #7487, 1000.000000000000000 ) ;
#6441=EDGE_CURVE ( 'NONE', #4775, #4975, #1700, .T. ) ;
#6452=DIRECTION ( 'NONE',  ( 1.000000000000000000, 2.715219353702832714E-15, 0.000000000000000000 ) ) ;
#6469=DIRECTION ( 'NONE',  ( 1.000000000000000000, 3.083952846180994816E-15, 0.000000000000000000 ) ) ;
#6472=DIRECTION ( 'NONE',  ( -3.919652622816902408E-30, -3.944304526105059027E-30, 1.000000000000000000 ) ) ;
#6477=ORIENTED_EDGE ( 'NONE', *, *, #1626, .T. ) ;
#6486=DIRECTION ( 'NONE',  ( -1.000000000000000000, -3.083952846180997183E-15, 0.000000000000000000 ) ) ;
#6497=VERTEX_POINT ( 'NONE', #7928 ) ;
#6508=AXIS2_PLACEMENT_3D ( 'NONE', #2865, #1633, #6322 ) ;
#6514=( LENGTH_UNIT ( ) NAMED_UNIT ( * ) SI_UNIT ( .MILLI., .METRE. ) );
#6515=ORIENTED_EDGE ( 'NONE', *, *, #5016, .F. ) ;
#6558=ORIENTED_EDGE ( 'NONE', *, *, #2194, .T. ) ;
#6561=CIRCLE ( 'NONE', #7958, 4.499999999999983125 ) ;
#6590=CARTESIAN_POINT ( 'NONE',  ( -17.49999999999955236, 120.0000000000003268, 9.999999999999980460 ) ) ;
#6603=DIRECTION ( 'NONE',  ( -1.000000000000000000, -2.715219353702832714E-15, 0.000000000000000000 ) ) ;
#6605=FACE_BOUND ( 'NONE', #5501, .T. ) ;
#6614=CARTESIAN_POINT ( 'NONE',  ( -25.74999999999982947, 15.00000000000010836, 10.00000000000000888 ) ) ;
#6620=ORIENTED_EDGE ( 'NONE', *, *, #6441, .F. ) ;
#6636=VERTEX_POINT ( 'NONE', #1641 ) ;
#6641=DIRECTION ( 'NONE',  ( -3.919652622816902408E-30, -3.944304526105059027E-30, 1.000000000000000000 ) ) ;
#6673=CARTESIAN_POINT ( 'NONE',  ( -64.99999999999944578, 120.0000000000002842, 9.999999999999980460 ) ) ;
#6683=AXIS2_PLACEMENT_3D ( 'NONE', #6590, #1883, #5377 ) ;
#6686=AXIS2_PLACEMENT_3D ( 'NONE', #3856, #5893, #437 ) ;
#6687=CARTESIAN_POINT ( 'NONE',  ( 0.000000000000000000, 0.000000000000000000, 10.00000000000000888 ) ) ;
#6694=DIRECTION ( 'NONE',  ( -3.919652622816902408E-30, -3.944304526105059027E-30, 1.000000000000000000 ) ) ;
#6717=EDGE_LOOP ( 'NONE', ( #6996, #2729, #2577, #5026 ) ) ;
#6725=EDGE_CURVE ( 'NONE', #484, #2264, #5851, .T. ) ;
#6727=CARTESIAN_POINT ( 'NONE',  ( -64.99999999999945999, 120.0000000000002842, -5.879478934225335676E-29 ) ) ;
#6728=ORIENTED_EDGE ( 'NONE', *, *, #672, .T. ) ;
#6734=FACE_OUTER_BOUND ( 'NONE', #1607, .T. ) ;
#6742=ORIENTED_EDGE ( 'NONE', *, *, #5598, .T. ) ;
#6755=CARTESIAN_POINT ( 'NONE',  ( -99.99999999999972999, 0.000000000000000000, 9.999999999999980460 ) ) ;
#6765=CYLINDRICAL_SURFACE ( 'NONE', #3091, 4.499999999999993783 ) ;
#6773=EDGE_CURVE ( 'NONE', #5363, #5659, #5855, .T. ) ;
#6784=CARTESIAN_POINT ( 'NONE',  ( -49.99999999999953815, 120.0000000000003268, 9.999999999999980460 ) ) ;
#6791=DIRECTION ( 'NONE',  ( -1.000000000000000000, -2.775557561562891745E-15, 0.000000000000000000 ) ) ;
#6801=ORIENTED_EDGE ( 'NONE', *, *, #7891, .F. ) ;
#6810=VECTOR ( 'NONE', #6882, 1000.000000000000000 ) ;
#6818=DIRECTION ( 'NONE',  ( -3.919652622816902408E-30, -3.944304526105059027E-30, 1.000000000000000000 ) ) ;
#6823=ORIENTED_EDGE ( 'NONE', *, *, #6725, .T. ) ;
#6827=CARTESIAN_POINT ( 'NONE',  ( -49.99999999999949551, 152.5000000000003126, -1.942890293094023946E-13 ) ) ;
#6832=EDGE_CURVE ( 'NONE', #4975, #4775, #3044, .T. ) ;
#6847=ADVANCED_FACE ( 'NONE', ( #4789 ), #3393, .F. ) ;
#6856=LINE ( 'NONE', #5463, #6280 ) ;
#6877=EDGE_CURVE ( 'NONE', #683, #4883, #8058, .T. ) ;
#6882=DIRECTION ( 'NONE',  ( 1.000000000000000000, 2.775557561562898056E-15, -3.821045009664285041E-30 ) ) ;
#6912=EDGE_LOOP ( 'NONE', ( #5881, #6742 ) ) ;
#6921=CARTESIAN_POINT ( 'NONE',  ( -17.49999999999958078, 120.0000000000003268, 0.000000000000000000 ) ) ;
#6944=AXIS2_PLACEMENT_3D ( 'NONE', #3825, #7786, #5044 ) ;
#6965=CARTESIAN_POINT ( 'NONE',  ( 4.059252933785728601E-13, 119.9999999999998863, 10.00000000000000888 ) ) ;
#6979=AXIS2_PLACEMENT_3D ( 'NONE', #3288, #2643, #3990 ) ;
#6986=ADVANCED_FACE ( 'NONE', ( #8271 ), #3610, .F. ) ;
#6996=ORIENTED_EDGE ( 'NONE', *, *, #3230, .T. ) ;
#7002=VECTOR ( 'NONE', #1803, 1000.000000000000000 ) ;
#7012=CARTESIAN_POINT ( 'NONE',  ( -77.99999999999947420, 120.0000000000003411, 10.00000000000000888 ) ) ;
#7037=VERTEX_POINT ( 'NONE', #2334 ) ;
#7040=EDGE_CURVE ( 'NONE', #4829, #704, #7615, .T. ) ;
#7050=DIRECTION ( 'NONE',  ( 1.000000000000000000, -1.619075244245011343E-15, -3.722437396511636845E-30 ) ) ;
#7066=ORIENTED_EDGE ( 'NONE', *, *, #8354, .F. ) ;
#7073=EDGE_CURVE ( 'NONE', #1650, #5363, #910, .T. ) ;
#7078=LINE ( 'NONE', #1107, #7002 ) ;
#7088=APPLICATION_CONTEXT ( 'automotive_design' ) ;
#7092=ORIENTED_EDGE ( 'NONE', *, *, #2663, .F. ) ;
#7117=ORIENTED_EDGE ( 'NONE', *, *, #5705, .F. ) ;
#7118=CARTESIAN_POINT ( 'NONE',  ( -45.49999999999946709, 152.5000000000003126, 9.999999999999786837 ) ) ;
#7157=DIRECTION ( 'NONE',  ( -3.919652622816902408E-30, -3.944304526105059027E-30, 1.000000000000000000 ) ) ;
#7158=ORIENTED_EDGE ( 'NONE', *, *, #7761, .T. ) ;
#7160=ADVANCED_FACE ( 'NONE', ( #472 ), #7816, .F. ) ;
#7184=EDGE_CURVE ( 'NONE', #2953, #5659, #4346, .T. ) ;
#7187=EDGE_LOOP ( 'NONE', ( #7526, #6477 ) ) ;
#7189=VERTEX_POINT ( 'NONE', #3817 ) ;
#7194=ORIENTED_EDGE ( 'NONE', *, *, #6043, .F. ) ;
#7222=VERTEX_POINT ( 'NONE', #1157 ) ;
#7227=ORIENTED_EDGE ( 'NONE', *, *, #7040, .T. ) ;
#7251=DIRECTION ( 'NONE',  ( 3.498359009886546906E-15, 1.000000000000000000, -3.747089299799789961E-30 ) ) ;
#7261=DIRECTION ( 'NONE',  ( -3.919652622816902408E-30, -3.944304526105059027E-30, 1.000000000000000000 ) ) ;
#7270=SHAPE_REPRESENTATION ( 'Motor mount pad', ( #7563 ), #2705 ) ;
#7289=ORIENTED_EDGE ( 'NONE', *, *, #7626, .F. ) ;
#7320=CIRCLE ( 'NONE', #642, 4.499999999999993783 ) ;
#7335=EDGE_CURVE ( 'NONE', #1650, #2953, #4439, .T. ) ;
#7362=ORIENTED_EDGE ( 'NONE', *, *, #1626, .F. ) ;
#7386=CARTESIAN_POINT ( 'NONE',  ( -79.99999999999972999, 15.00000000000012434, 1.942890293094023946E-13 ) ) ;
#7393=DIRECTION ( 'NONE',  ( -1.619075244245011540E-15, -1.000000000000000000, 3.747089299799789961E-30 ) ) ;
#7413=EDGE_CURVE ( 'NONE', #757, #6636, #548, .T. ) ;
#7415=VECTOR ( 'NONE', #8433, 1000.000000000000000 ) ;
#7425=DIRECTION ( 'NONE',  ( 1.000000000000000000, 3.083952846180994816E-15, 0.000000000000000000 ) ) ;
#7431=ORIENTED_EDGE ( 'NONE', *, *, #3430, .F. ) ;
#7473=DIRECTION ( 'NONE',  ( -1.000000000000000000, -2.775557561562916200E-15, 0.000000000000000000 ) ) ;
#7478=DIRECTION ( 'NONE',  ( 0.000000000000000000, 0.000000000000000000, 1.000000000000000000 ) ) ;
#7483=ORIENTED_EDGE ( 'NONE', *, *, #8339, .T. ) ;
#7484=EDGE_CURVE ( 'NONE', #6113, #4846, #4942, .T. ) ;
#7487=DIRECTION ( 'NONE',  ( 3.919652622816902408E-30, 3.944304526105059027E-30, -1.000000000000000000 ) ) ;
#7516=CLOSED_SHELL ( 'NONE', ( #7850, #7709, #439, #2942, #6986, #8159, #3785, #3043, #5532, #3561, #522, #5616, #8447, #5938, #6847, #7160, #4143, #2166, #2017, #4810 ) ) ;
#7523=( GEOMETRIC_REPRESENTATION_CONTEXT ( 3 ) GLOBAL_UNCERTAINTY_ASSIGNED_CONTEXT ( ( #357 ) ) GLOBAL_UNIT_ASSIGNED_CONTEXT ( ( #6514, #8514, #2558 ) ) REPRESENTATION_CONTEXT ( 'NONE', 'WORKASPACE' ) );
#7526=ORIENTED_EDGE ( 'NONE', *, *, #6773, .T. ) ;
#7527=LINE ( 'NONE', #1550, #178 ) ;
#7531=LINE ( 'NONE', #6197, #7565 ) ;
#7540=ORIENTED_EDGE ( 'NONE', *, *, #1227, .T. ) ;
#7551=ORIENTED_EDGE ( 'NONE', *, *, #6877, .T. ) ;
#7563=AXIS2_PLACEMENT_3D ( 'NONE', #4203, #7478, #3512 ) ;
#7565=VECTOR ( 'NONE', #2867, 1000.000000000000000 ) ;
#7573=DIRECTION ( 'NONE',  ( -3.919652622816902408E-30, -3.944304526105059027E-30, 1.000000000000000000 ) ) ;
#7611=PLANE ( 'NONE',  #6238 ) ;
#7615=LINE ( 'NONE', #6153, #6810 ) ;
#7617=EDGE_LOOP ( 'NONE', ( #5595, #6801 ) ) ;
#7626=EDGE_CURVE ( 'NONE', #2216, #605, #5708, .T. ) ;
#7637=EDGE_LOOP ( 'NONE', ( #6133, #5023 ) ) ;
#7669=DIRECTION ( 'NONE',  ( 1.000000000000000000, 2.775557561562892140E-15, -3.821045009664285742E-30 ) ) ;
#7681=CARTESIAN_POINT ( 'NONE',  ( -12.99999999999955058, 120.0000000000003411, 9.999999999999980460 ) ) ;
#7688=ORIENTED_EDGE ( 'NONE', *, *, #647, .T. ) ;
#7696=APPLICATION_CONTEXT ( 'automotive_design' ) ;
#7709=ADVANCED_FACE ( 'NONE', ( #5022 ), #4457, .F. ) ;
#7710=EDGE_CURVE ( 'NONE', #4975, #757, #3066, .T. ) ;
#7723=ORIENTED_EDGE ( 'NONE', *, *, #165, .F. ) ;
#7732=DIRECTION ( 'NONE',  ( -1.000000000000000000, 0.000000000000000000, 0.000000000000000000 ) ) ;
#7747=DIRECTION ( 'NONE',  ( -3.919652622816902408E-30, -3.944304526105059027E-30, 1.000000000000000000 ) ) ;
#7760=CARTESIAN_POINT ( 'NONE',  ( 0.000000000000000000, 0.000000000000000000, 0.000000000000000000 ) ) ;
#7761=EDGE_CURVE ( 'NONE', #7222, #7833, #5879, .T. ) ;
#7786=DIRECTION ( 'NONE',  ( -3.919652622816902408E-30, -3.944304526105059027E-30, 1.000000000000000000 ) ) ;
#7794=CYLINDRICAL_SURFACE ( 'NONE', #8314, 4.499999999999990230 ) ;
#7799=LINE ( 'NONE', #365, #2780 ) ;
#7801=EDGE_CURVE ( 'NONE', #605, #4429, #3884, .T. ) ;
#7816=CYLINDRICAL_SURFACE ( 'NONE', #3183, 4.499999999999983125 ) ;
#7817=DIRECTION ( 'NONE',  ( 1.000000000000000000, 2.775557561562898056E-15, -3.821045009664285041E-30 ) ) ;
#7823=CIRCLE ( 'NONE', #320, 4.499999999999997335 ) ;
#7829=CARTESIAN_POINT ( 'NONE',  ( -49.99999999999944578, 152.5000000000003126, 9.999999999999786837 ) ) ;
#7833=VERTEX_POINT ( 'NONE', #575 ) ;
#7845=DIRECTION ( 'NONE',  ( -1.000000000000000000, -2.715219353702835870E-15, 0.000000000000000000 ) ) ;
#7846=CYLINDRICAL_SURFACE ( 'NONE', #6683, 4.499999999999993783 ) ;
#7850=ADVANCED_FACE ( 'NONE', ( #3232 ), #1323, .F. ) ;
#7864=ORIENTED_EDGE ( 'NONE', *, *, #6043, .T. ) ;
#7891=EDGE_CURVE ( 'NONE', #2953, #1650, #5580, .T. ) ;
#7906=LINE ( 'NONE', #4652, #1299 ) ;
#7916=DIRECTION ( 'NONE',  ( -3.919652622816902408E-30, -3.944304526105059027E-30, 1.000000000000000000 ) ) ;
#7925=CARTESIAN_POINT ( 'NONE',  ( -34.99999999999963762, 120.0000000000003695, 5.879478934225333434E-29 ) ) ;
#7928=CARTESIAN_POINT ( 'NONE',  ( -99.99999999999958789, 120.0000000000001137, 0.000000000000000000 ) ) ;
#7943=EDGE_CURVE ( 'NONE', #4252, #3370, #2921, .T. ) ;
#7945=ORIENTED_EDGE ( 'NONE', *, *, #6877, .F. ) ;
#7949=CYLINDRICAL_SURFACE ( 'NONE', #8063, 5.749999999999991118 ) ;
#7958=AXIS2_PLACEMENT_3D ( 'NONE', #1194, #6472, #3162 ) ;
#7992=EDGE_CURVE ( 'NONE', #7037, #6198, #8481, .T. ) ;
#8001=EDGE_LOOP ( 'NONE', ( #117, #1732, #6346, #4955 ) ) ;
#8005=CARTESIAN_POINT ( 'NONE',  ( -77.99999999999941735, 120.0000000000003411, -2.775557561562889458E-14 ) ) ;
#8014=CIRCLE ( 'NONE', #4113, 14.99999999999987388 ) ;
#8020=DIRECTION ( 'NONE',  ( -1.000000000000000000, -3.083952846180994816E-15, 0.000000000000000000 ) ) ;
#8058=CIRCLE ( 'NONE', #407, 49.99999999999998579 ) ;
#8063=AXIS2_PLACEMENT_3D ( 'NONE', #5298, #6012, #6603 ) ;
#8073=AXIS2_PLACEMENT_3D ( 'NONE', #8379, #5146, #5830 ) ;
#8092=VECTOR ( 'NONE', #3874, 1000.000000000000000 ) ;
#8099=DIRECTION ( 'NONE',  ( 1.000000000000000000, 3.083952846180992055E-15, 0.000000000000000000 ) ) ;
#8120=CARTESIAN_POINT ( 'NONE',  ( -82.49999999999945999, 120.0000000000003268, 10.00000000000000888 ) ) ;
#8127=FACE_OUTER_BOUND ( 'NONE', #1706, .T. ) ;
#8134=FACE_BOUND ( 'NONE', #5714, .T. ) ;
#8138=CARTESIAN_POINT ( 'NONE',  ( -49.99999999999953815, 120.0000000000003268, 9.999999999999980460 ) ) ;
#8159=ADVANCED_FACE ( 'NONE', ( #1346 ), #1475, .F. ) ;
#8169=ORIENTED_EDGE ( 'NONE', *, *, #3516, .F. ) ;
#8172=FACE_OUTER_BOUND ( 'NONE', #5653, .T. ) ;
#8173=ORIENTED_EDGE ( 'NONE', *, *, #165, .T. ) ;
#8191=AXIS2_PLACEMENT_3D ( 'NONE', #5734, #8443, #8364 ) ;
#8200=AXIS2_PLACEMENT_3D ( 'NONE', #1788, #2404, #3301 ) ;
#8209=EDGE_CURVE ( 'NONE', #7222, #4804, #2289, .T. ) ;
#8214=VECTOR ( 'NONE', #328, 1000.000000000000000 ) ;
#8225=FACE_OUTER_BOUND ( 'NONE', #5246, .T. ) ;
#8229=CARTESIAN_POINT ( 'NONE',  ( -79.99999999999980105, 15.00000000000012434, 10.00000000000017586 ) ) ;
#8262=VECTOR ( 'NONE', #751, 1000.000000000000000 ) ;
#8271=FACE_OUTER_BOUND ( 'NONE', #4645, .T. ) ;
#8314=AXIS2_PLACEMENT_3D ( 'NONE', #658, #3135, #6486 ) ;
#8320=ORIENTED_EDGE ( 'NONE', *, *, #8354, .T. ) ;
#8339=EDGE_CURVE ( 'NONE', #4775, #6636, #7531, .T. ) ;
#8349=CARTESIAN_POINT ( 'NONE',  ( 0.000000000000000000, 0.000000000000000000, 10.00000000000000888 ) ) ;
#8354=EDGE_CURVE ( 'NONE', #6000, #2499, #5400, .T. ) ;
#8364=DIRECTION ( 'NONE',  ( 1.000000000000000000, 3.083952846180997183E-15, -4.108650548026112028E-30 ) ) ;
#8379=CARTESIAN_POINT ( 'NONE',  ( -49.99999999999963762, 87.50000000000035527, 9.999999999999786837 ) ) ;
#8398=ORIENTED_EDGE ( 'NONE', *, *, #5342, .T. ) ;
#8433=DIRECTION ( 'NONE',  ( 3.919652622816902408E-30, 3.944304526105059027E-30, -1.000000000000000000 ) ) ;
#8438=CARTESIAN_POINT ( 'NONE',  ( -99.99999999999972999, 0.000000000000000000, 9.999999999999980460 ) ) ;
#8443=DIRECTION ( 'NONE',  ( -3.919652622816902408E-30, -3.944304526105059027E-30, 1.000000000000000000 ) ) ;
#8447=ADVANCED_FACE ( 'NONE', ( #3123 ), #5808, .F. ) ;
#8472=FACE_BOUND ( 'NONE', #7187, .T. ) ;
#8481=CIRCLE ( 'NONE', #2110, 4.499999999999993783 ) ;
#8514=( NAMED_UNIT ( * ) PLANE_ANGLE_UNIT ( ) SI_UNIT ( $, .RADIAN. ) );
#8525=CIRCLE ( 'NONE', #336, 5.749999999999985789 ) ;
#8548=PRODUCT_DEFINITION_CONTEXT ( 'detailed design', #7088, 'design' ) ;
#8560=AXIS2_PLACEMENT_3D ( 'NONE', #2173, #59, #6791 ) ;
#8578=EDGE_LOOP ( 'NONE', ( #6038, #1564, #4570, #4542 ) ) ;
#8586=EDGE_CURVE ( 'NONE', #4804, #7189, #7906, .T. ) ;
#8598=FACE_BOUND ( 'NONE', #6912, .T. ) ;
#8650=COLOUR_RGB('Sky Blue',0.24,0.69,0.87);
#8651=FILL_AREA_STYLE_COLOUR('',#8650);
#8652=FILL_AREA_STYLE('',(#8651));
#8653=SURFACE_STYLE_FILL_AREA(#8652);
#8654=SURFACE_SIDE_STYLE('',(#8653));
#8655=SURFACE_STYLE_USAGE(.BOTH.,#8654);
#8656=PRESENTATION_STYLE_ASSIGNMENT((#8655));
ENDSEC;
END-ISO-10303-21;
